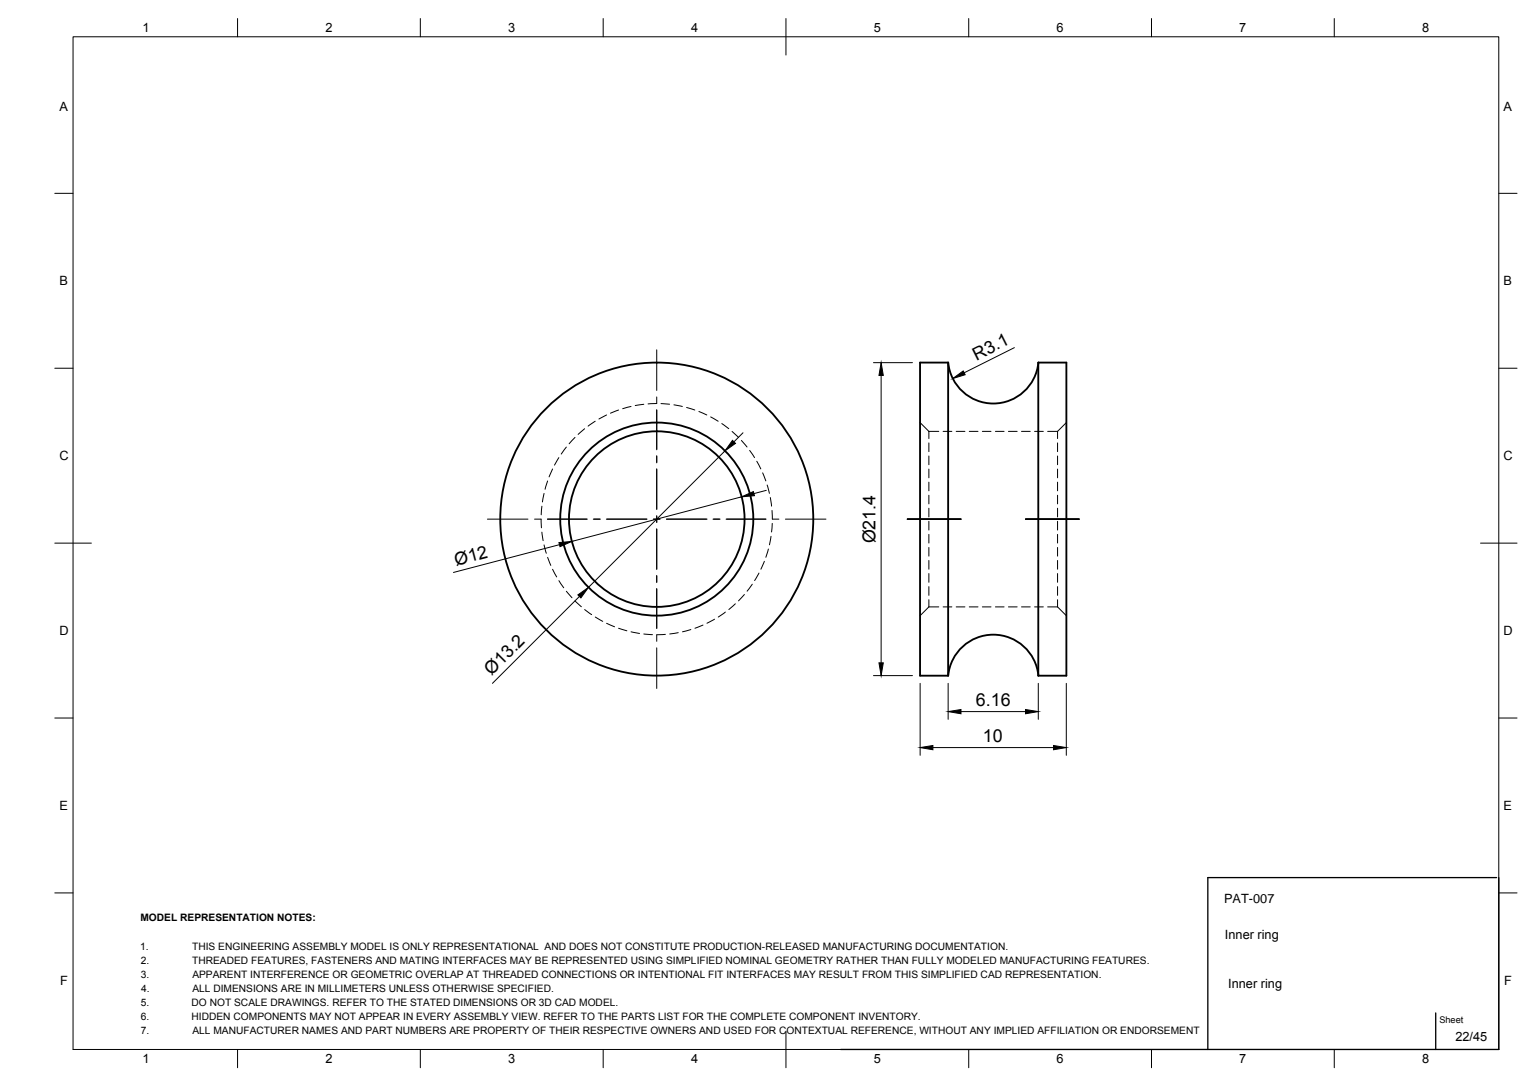
ISO-10303-21;
HEADER;
/* Generated by software containing ST-Developer
 * from STEP Tools, Inc. (www.steptools.com) 
 */

FILE_DESCRIPTION(
/* description */ ('Bearing friction torque test rig'),
/* implementation_level */ '2;1');

FILE_NAME(
/* name */ 'Inner ring.step',
/* time_stamp */ '2026-10-28T03:24:04-07:00',
/* author */ (''),
/* organization */ (''),
/* preprocessor_version */ 'ST-DEVELOPER v20.2',
/* originating_system */ 'Autodesk Translation Framework v15.17.0.0',
/* authorisation */ '');

FILE_SCHEMA (('AUTOMOTIVE_DESIGN { 1 0 10303 214 3 1 1 }'));
ENDSEC;

DATA;
#10=MECHANICAL_DESIGN_GEOMETRIC_PRESENTATION_REPRESENTATION('',(#555),#14822);
#425=TOROIDAL_SURFACE('',#8624,1.1,0.309556);
#432=CONICAL_SURFACE('',#8635,0.63,0.785398163397448);
#433=CONICAL_SURFACE('',#8642,0.63,0.785398163397448);
#477=SHAPE_REPRESENTATION_RELATIONSHIP('SRR','None',#15017,#516);
#516=ADVANCED_BREP_SHAPE_REPRESENTATION('',(#608),#14797);
#555=STYLED_ITEM('',(#15284),#608);
#608=MANIFOLD_SOLID_BREP('Body1',#7672);
#814=FACE_BOUND('',#1956,.T.);
#815=FACE_BOUND('',#1959,.T.);
#1002=PLANE('',#8637);
#1003=PLANE('',#8640);
#1336=FACE_OUTER_BOUND('',#1951,.T.);
#1337=FACE_OUTER_BOUND('',#1952,.T.);
#1338=FACE_OUTER_BOUND('',#1953,.T.);
#1339=FACE_OUTER_BOUND('',#1954,.T.);
#1340=FACE_OUTER_BOUND('',#1955,.T.);
#1341=FACE_OUTER_BOUND('',#1957,.T.);
#1342=FACE_OUTER_BOUND('',#1958,.T.);
#1343=FACE_OUTER_BOUND('',#1960,.T.);
#1951=EDGE_LOOP('',(#6204,#6205,#6206,#6207,#6208,#6209));
#1952=EDGE_LOOP('',(#6210,#6211,#6212,#6213,#6214));
#1953=EDGE_LOOP('',(#6215,#6216,#6217,#6218));
#1954=EDGE_LOOP('',(#6219,#6220,#6221,#6222));
#1955=EDGE_LOOP('',(#6223));
#1956=EDGE_LOOP('',(#6224));
#1957=EDGE_LOOP('',(#6225,#6226,#6227,#6228,#6229));
#1958=EDGE_LOOP('',(#6230));
#1959=EDGE_LOOP('',(#6231));
#1960=EDGE_LOOP('',(#6232,#6233,#6234,#6235));
#2522=LINE('',#12806,#2966);
#2523=LINE('',#12812,#2967);
#2524=LINE('',#12816,#2968);
#2525=LINE('',#12822,#2969);
#2526=LINE('',#12827,#2970);
#2966=VECTOR('',#10447,1.070235);
#2967=VECTOR('',#10454,0.6);
#2968=VECTOR('',#10459,0.63);
#2969=VECTOR('',#10468,1.070235);
#2970=VECTOR('',#10475,0.63);
#3326=CIRCLE('',#8625,1.070235);
#3327=CIRCLE('',#8626,1.070235);
#3328=CIRCLE('',#8627,0.309556);
#3329=CIRCLE('',#8628,1.070235);
#3330=CIRCLE('',#8629,1.070235);
#3331=CIRCLE('',#8631,1.070235);
#3332=CIRCLE('',#8633,0.6);
#3333=CIRCLE('',#8634,0.6);
#3334=CIRCLE('',#8636,0.66);
#3335=CIRCLE('',#8639,1.070235);
#3336=CIRCLE('',#8641,0.66);
#3904=VERTEX_POINT('',#12795);
#3905=VERTEX_POINT('',#12796);
#3906=VERTEX_POINT('',#12799);
#3907=VERTEX_POINT('',#12801);
#3908=VERTEX_POINT('',#12805);
#3909=VERTEX_POINT('',#12809);
#3910=VERTEX_POINT('',#12811);
#3911=VERTEX_POINT('',#12815);
#3912=VERTEX_POINT('',#12820);
#3913=VERTEX_POINT('',#12824);
#4728=EDGE_CURVE('',#3904,#3905,#3326,.T.);
#4729=EDGE_CURVE('',#3905,#3904,#3327,.T.);
#4730=EDGE_CURVE('',#3905,#3906,#3328,.T.);
#4731=EDGE_CURVE('',#3907,#3906,#3329,.T.);
#4732=EDGE_CURVE('',#3906,#3907,#3330,.T.);
#4733=EDGE_CURVE('',#3907,#3908,#2522,.T.);
#4734=EDGE_CURVE('',#3908,#3908,#3331,.T.);
#4735=EDGE_CURVE('',#3909,#3909,#3332,.T.);
#4736=EDGE_CURVE('',#3909,#3910,#2523,.T.);
#4737=EDGE_CURVE('',#3910,#3910,#3333,.T.);
#4738=EDGE_CURVE('',#3910,#3911,#2524,.T.);
#4739=EDGE_CURVE('',#3911,#3911,#3334,.T.);
#4740=EDGE_CURVE('',#3912,#3912,#3335,.T.);
#4741=EDGE_CURVE('',#3912,#3904,#2525,.T.);
#4742=EDGE_CURVE('',#3913,#3913,#3336,.T.);
#4743=EDGE_CURVE('',#3913,#3909,#2526,.T.);
#6204=ORIENTED_EDGE('',*,*,#4728,.F.);
#6205=ORIENTED_EDGE('',*,*,#4729,.F.);
#6206=ORIENTED_EDGE('',*,*,#4730,.T.);
#6207=ORIENTED_EDGE('',*,*,#4731,.F.);
#6208=ORIENTED_EDGE('',*,*,#4732,.F.);
#6209=ORIENTED_EDGE('',*,*,#4730,.F.);
#6210=ORIENTED_EDGE('',*,*,#4731,.T.);
#6211=ORIENTED_EDGE('',*,*,#4732,.T.);
#6212=ORIENTED_EDGE('',*,*,#4733,.T.);
#6213=ORIENTED_EDGE('',*,*,#4734,.T.);
#6214=ORIENTED_EDGE('',*,*,#4733,.F.);
#6215=ORIENTED_EDGE('',*,*,#4735,.T.);
#6216=ORIENTED_EDGE('',*,*,#4736,.T.);
#6217=ORIENTED_EDGE('',*,*,#4737,.F.);
#6218=ORIENTED_EDGE('',*,*,#4736,.F.);
#6219=ORIENTED_EDGE('',*,*,#4737,.T.);
#6220=ORIENTED_EDGE('',*,*,#4738,.T.);
#6221=ORIENTED_EDGE('',*,*,#4739,.F.);
#6222=ORIENTED_EDGE('',*,*,#4738,.F.);
#6223=ORIENTED_EDGE('',*,*,#4734,.F.);
#6224=ORIENTED_EDGE('',*,*,#4739,.T.);
#6225=ORIENTED_EDGE('',*,*,#4740,.F.);
#6226=ORIENTED_EDGE('',*,*,#4741,.T.);
#6227=ORIENTED_EDGE('',*,*,#4728,.T.);
#6228=ORIENTED_EDGE('',*,*,#4729,.T.);
#6229=ORIENTED_EDGE('',*,*,#4741,.F.);
#6230=ORIENTED_EDGE('',*,*,#4740,.T.);
#6231=ORIENTED_EDGE('',*,*,#4742,.F.);
#6232=ORIENTED_EDGE('',*,*,#4742,.T.);
#6233=ORIENTED_EDGE('',*,*,#4743,.T.);
#6234=ORIENTED_EDGE('',*,*,#4735,.F.);
#6235=ORIENTED_EDGE('',*,*,#4743,.F.);
#7150=CYLINDRICAL_SURFACE('',#8630,1.070235);
#7151=CYLINDRICAL_SURFACE('',#8632,0.6);
#7152=CYLINDRICAL_SURFACE('',#8638,1.070235);
#7447=ADVANCED_FACE('',(#1336),#425,.F.);
#7448=ADVANCED_FACE('',(#1337),#7150,.T.);
#7449=ADVANCED_FACE('',(#1338),#7151,.F.);
#7450=ADVANCED_FACE('',(#1339),#432,.F.);
#7451=ADVANCED_FACE('',(#1340,#814),#1002,.T.);
#7452=ADVANCED_FACE('',(#1341),#7152,.T.);
#7453=ADVANCED_FACE('',(#1342,#815),#1003,.T.);
#7454=ADVANCED_FACE('',(#1343),#433,.F.);
#7672=CLOSED_SHELL('',(#7447,#7448,#7449,#7450,#7451,#7452,#7453,#7454));
#8623=AXIS2_PLACEMENT_3D('',#12793,#10431,#10432);
#8624=AXIS2_PLACEMENT_3D('',#12794,#10433,#10434);
#8625=AXIS2_PLACEMENT_3D('',#12797,#10435,#10436);
#8626=AXIS2_PLACEMENT_3D('',#12798,#10437,#10438);
#8627=AXIS2_PLACEMENT_3D('',#12800,#10439,#10440);
#8628=AXIS2_PLACEMENT_3D('',#12802,#10441,#10442);
#8629=AXIS2_PLACEMENT_3D('',#12803,#10443,#10444);
#8630=AXIS2_PLACEMENT_3D('',#12804,#10445,#10446);
#8631=AXIS2_PLACEMENT_3D('',#12807,#10448,#10449);
#8632=AXIS2_PLACEMENT_3D('',#12808,#10450,#10451);
#8633=AXIS2_PLACEMENT_3D('',#12810,#10452,#10453);
#8634=AXIS2_PLACEMENT_3D('',#12813,#10455,#10456);
#8635=AXIS2_PLACEMENT_3D('',#12814,#10457,#10458);
#8636=AXIS2_PLACEMENT_3D('',#12817,#10460,#10461);
#8637=AXIS2_PLACEMENT_3D('',#12818,#10462,#10463);
#8638=AXIS2_PLACEMENT_3D('',#12819,#10464,#10465);
#8639=AXIS2_PLACEMENT_3D('',#12821,#10466,#10467);
#8640=AXIS2_PLACEMENT_3D('',#12823,#10469,#10470);
#8641=AXIS2_PLACEMENT_3D('',#12825,#10471,#10472);
#8642=AXIS2_PLACEMENT_3D('',#12826,#10473,#10474);
#10431=DIRECTION('axis',(0.,0.,1.));
#10432=DIRECTION('refdir',(1.,0.,0.));
#10433=DIRECTION('center_axis',(0.,-1.,0.));
#10434=DIRECTION('ref_axis',(0.,0.,-1.));
#10435=DIRECTION('center_axis',(0.,-1.,0.));
#10436=DIRECTION('ref_axis',(1.,0.,0.));
#10437=DIRECTION('center_axis',(0.,-1.,0.));
#10438=DIRECTION('ref_axis',(1.,0.,0.));
#10439=DIRECTION('center_axis',(1.,0.,1.22464679914735E-16));
#10440=DIRECTION('ref_axis',(-1.22464679914735E-16,0.,1.));
#10441=DIRECTION('center_axis',(0.,1.,0.));
#10442=DIRECTION('ref_axis',(1.,0.,0.));
#10443=DIRECTION('center_axis',(0.,1.,0.));
#10444=DIRECTION('ref_axis',(1.,0.,0.));
#10445=DIRECTION('center_axis',(0.,-1.,0.));
#10446=DIRECTION('ref_axis',(1.,0.,0.));
#10447=DIRECTION('',(0.,1.,0.));
#10448=DIRECTION('center_axis',(0.,-1.,0.));
#10449=DIRECTION('ref_axis',(1.,0.,0.));
#10450=DIRECTION('center_axis',(0.,-1.,0.));
#10451=DIRECTION('ref_axis',(1.,0.,0.));
#10452=DIRECTION('center_axis',(0.,-1.,0.));
#10453=DIRECTION('ref_axis',(1.,0.,0.));
#10454=DIRECTION('',(0.,1.,0.));
#10455=DIRECTION('center_axis',(0.,-1.,0.));
#10456=DIRECTION('ref_axis',(1.,0.,0.));
#10457=DIRECTION('center_axis',(0.,1.,0.));
#10458=DIRECTION('ref_axis',(1.,0.,0.));
#10459=DIRECTION('',(-0.707106781186548,0.707106781186547,-8.65956056235493E-17));
#10460=DIRECTION('center_axis',(0.,-1.,0.));
#10461=DIRECTION('ref_axis',(1.,0.,0.));
#10462=DIRECTION('center_axis',(0.,1.,0.));
#10463=DIRECTION('ref_axis',(0.,0.,1.));
#10464=DIRECTION('center_axis',(0.,-1.,0.));
#10465=DIRECTION('ref_axis',(1.,0.,0.));
#10466=DIRECTION('center_axis',(0.,-1.,0.));
#10467=DIRECTION('ref_axis',(1.,0.,0.));
#10468=DIRECTION('',(0.,1.,0.));
#10469=DIRECTION('center_axis',(0.,-1.,0.));
#10470=DIRECTION('ref_axis',(0.,0.,-1.));
#10471=DIRECTION('center_axis',(0.,-1.,0.));
#10472=DIRECTION('ref_axis',(1.,0.,0.));
#10473=DIRECTION('center_axis',(0.,-1.,0.));
#10474=DIRECTION('ref_axis',(1.,0.,0.));
#10475=DIRECTION('',(0.707106781186548,0.707106781186547,8.65956056235493E-17));
#12793=CARTESIAN_POINT('',(0.,0.,0.));
#12794=CARTESIAN_POINT('Origin',(0.,0.,0.));
#12795=CARTESIAN_POINT('',(-1.070235,-0.308121667383195,-1.31065986708547E-16));
#12796=CARTESIAN_POINT('',(-1.31065986708547E-16,-0.308121667383195,1.070235));
#12797=CARTESIAN_POINT('Origin',(0.,-0.308121667383195,0.));
#12798=CARTESIAN_POINT('Origin',(0.,-0.308121667383195,0.));
#12799=CARTESIAN_POINT('',(-1.31065986708547E-16,0.308121667383195,1.070235));
#12800=CARTESIAN_POINT('Origin',(-1.34711147906209E-16,0.,1.1));
#12801=CARTESIAN_POINT('',(-1.070235,0.308121667383195,1.31065986708547E-16));
#12802=CARTESIAN_POINT('Origin',(0.,0.308121667383195,0.));
#12803=CARTESIAN_POINT('Origin',(0.,0.308121667383195,0.));
#12804=CARTESIAN_POINT('Origin',(0.,0.,0.));
#12805=CARTESIAN_POINT('',(-1.070235,0.5,-1.31065986708547E-16));
#12806=CARTESIAN_POINT('',(-1.070235,0.,-1.31065986708547E-16));
#12807=CARTESIAN_POINT('Origin',(0.,0.5,0.));
#12808=CARTESIAN_POINT('Origin',(0.,0.,0.));
#12809=CARTESIAN_POINT('',(-0.6,-0.44,-7.34788079488412E-17));
#12810=CARTESIAN_POINT('Origin',(0.,-0.44,0.));
#12811=CARTESIAN_POINT('',(-0.6,0.44,-7.34788079488412E-17));
#12812=CARTESIAN_POINT('',(-0.6,0.,-7.34788079488412E-17));
#12813=CARTESIAN_POINT('Origin',(0.,0.44,0.));
#12814=CARTESIAN_POINT('Origin',(0.,0.47,0.));
#12815=CARTESIAN_POINT('',(-0.66,0.5,-8.08266887437253E-17));
#12816=CARTESIAN_POINT('',(-0.63,0.47,-7.71527483462832E-17));
#12817=CARTESIAN_POINT('Origin',(0.,0.5,0.));
#12818=CARTESIAN_POINT('Origin',(1.070235,0.5,0.));
#12819=CARTESIAN_POINT('Origin',(0.,0.,0.));
#12820=CARTESIAN_POINT('',(-1.070235,-0.5,-1.31065986708547E-16));
#12821=CARTESIAN_POINT('Origin',(0.,-0.5,0.));
#12822=CARTESIAN_POINT('',(-1.070235,0.,-1.31065986708547E-16));
#12823=CARTESIAN_POINT('Origin',(0.66,-0.5,0.));
#12824=CARTESIAN_POINT('',(-0.66,-0.5,-8.08266887437253E-17));
#12825=CARTESIAN_POINT('Origin',(0.,-0.5,0.));
#12826=CARTESIAN_POINT('Origin',(0.,-0.47,0.));
#12827=CARTESIAN_POINT('',(-0.63,-0.47,-7.71527483462832E-17));
#14752=UNCERTAINTY_MEASURE_WITH_UNIT(LENGTH_MEASURE(0.001),#14823,
'DISTANCE_ACCURACY_VALUE',
'Maximum model space distance between geometric entities at asserted c
onnectivities');
#14777=UNCERTAINTY_MEASURE_WITH_UNIT(LENGTH_MEASURE(0.001),#14823,
'DISTANCE_ACCURACY_VALUE',
'Maximum model space distance between geometric entities at asserted c
onnectivities');
#14797=(
GEOMETRIC_REPRESENTATION_CONTEXT(3)
GLOBAL_UNCERTAINTY_ASSIGNED_CONTEXT((#14752))
GLOBAL_UNIT_ASSIGNED_CONTEXT((#14823,#14825,#14826))
REPRESENTATION_CONTEXT('','3D')
);
#14822=(
GEOMETRIC_REPRESENTATION_CONTEXT(3)
GLOBAL_UNCERTAINTY_ASSIGNED_CONTEXT((#14777))
GLOBAL_UNIT_ASSIGNED_CONTEXT((#14823,#14825,#14826))
REPRESENTATION_CONTEXT('','3D')
);
#14823=(
LENGTH_UNIT()
NAMED_UNIT(*)
SI_UNIT(.CENTI.,.METRE.)
);
#14825=(
NAMED_UNIT(*)
PLANE_ANGLE_UNIT()
SI_UNIT($,.RADIAN.)
);
#14826=(
NAMED_UNIT(*)
SI_UNIT($,.STERADIAN.)
SOLID_ANGLE_UNIT()
);
#14846=SHAPE_DEFINITION_REPRESENTATION(#14890,#15017);
#14890=PRODUCT_DEFINITION_SHAPE('',$,#15062);
#15017=SHAPE_REPRESENTATION('',(#8623),#14797);
#15042=PRODUCT_DEFINITION_CONTEXT('part definition',#15176,'design');
#15062=PRODUCT_DEFINITION('Inner ring','Inner ring',#15106,#15042);
#15106=PRODUCT_DEFINITION_FORMATION('',$,#15197);
#15176=APPLICATION_CONTEXT(
'Core Data for Automotive Mechanical Design Process');
#15177=PRODUCT_CONTEXT('part definition',#15176,'mechanical');
#15197=PRODUCT('Inner ring','Inner ring','Inner ring',(#15177));
#15278=COLOUR_RGB('Grey',0.48,0.52,0.57);
#15279=FILL_AREA_STYLE_COLOUR('',#15278);
#15280=FILL_AREA_STYLE('',(#15279));
#15281=SURFACE_STYLE_FILL_AREA(#15280);
#15282=SURFACE_SIDE_STYLE('',(#15281));
#15283=SURFACE_STYLE_USAGE(.BOTH.,#15282);
#15284=PRESENTATION_STYLE_ASSIGNMENT((#15283));
ENDSEC;
END-ISO-10303-21;
